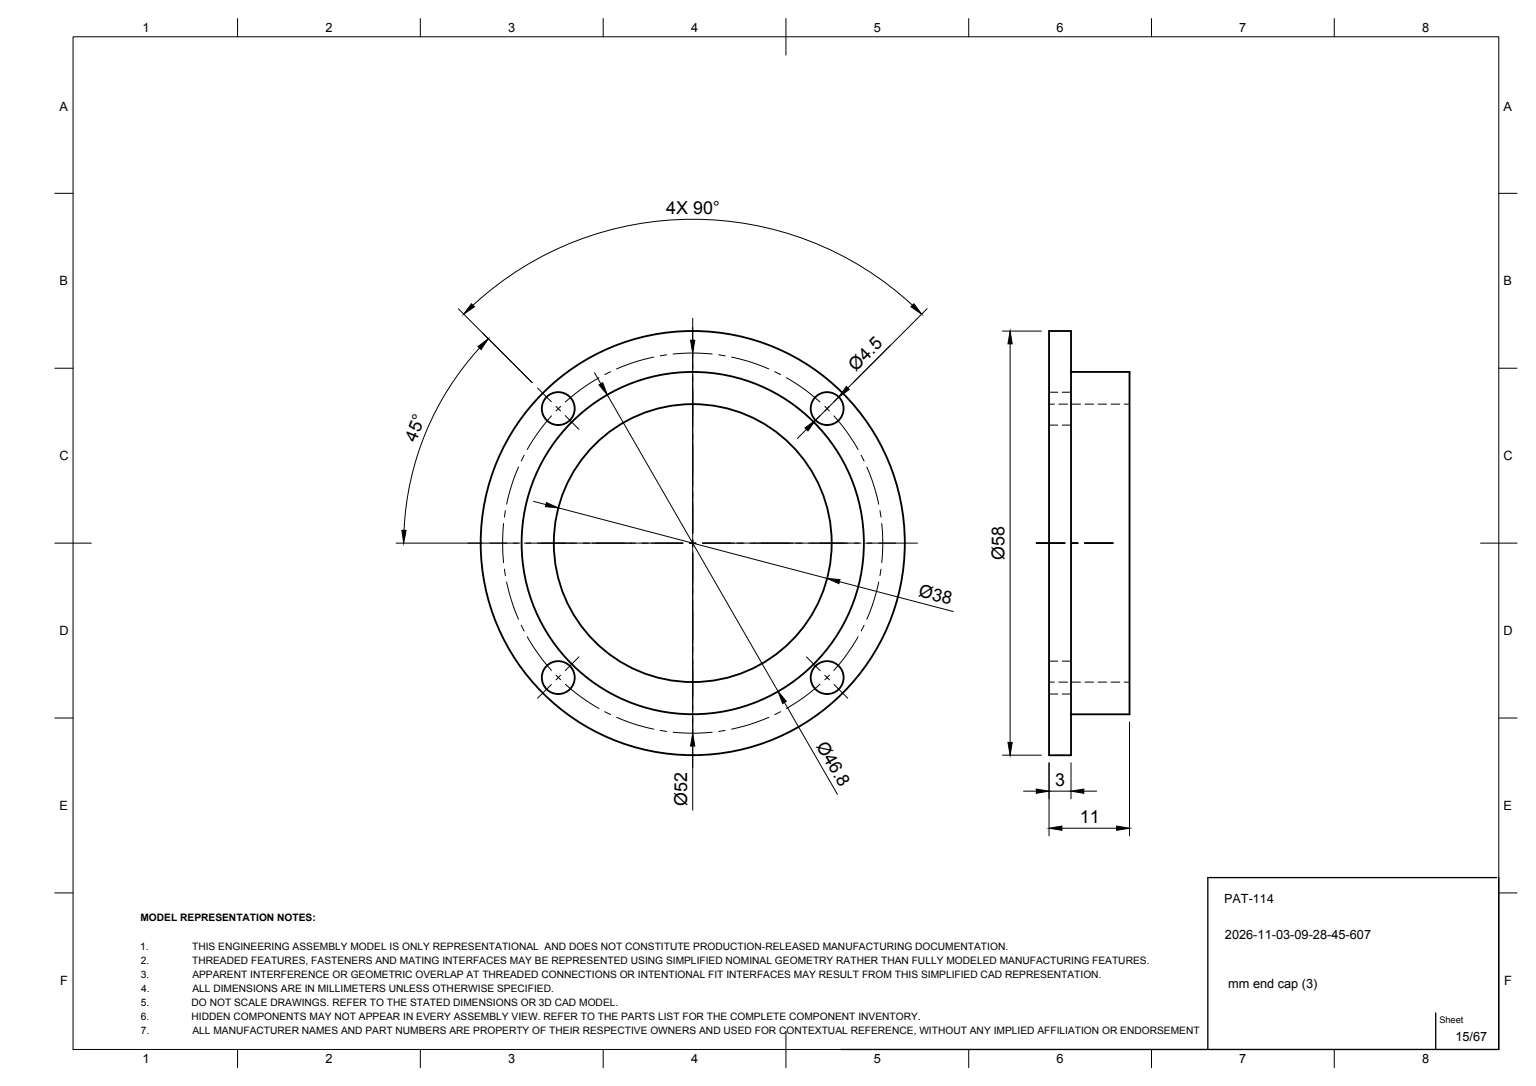
ISO-10303-21;
HEADER;
/* Generated by software containing ST-Developer
 * from STEP Tools, Inc. (www.steptools.com) 
 */

FILE_DESCRIPTION(
/* description */ ('Two-stage gear reducer in split housing'),
/* implementation_level */ '2;1');

FILE_NAME(
/* name */ 'mm end cap (3).step',
/* time_stamp */ '2026-10-28T03:22:31-07:00',
/* author */ (''),
/* organization */ (''),
/* preprocessor_version */ 'ST-DEVELOPER v20.2',
/* originating_system */ 'Autodesk Translation Framework v15.17.0.0',
/* authorisation */ '');

FILE_SCHEMA (('AUTOMOTIVE_DESIGN { 1 0 10303 214 3 1 1 }'));
ENDSEC;

DATA;
#10=MECHANICAL_DESIGN_GEOMETRIC_PRESENTATION_REPRESENTATION('',(#1244),#73366);
#1132=SHAPE_REPRESENTATION_RELATIONSHIP('SRR','None',#73619,#1188);
#1188=ADVANCED_BREP_SHAPE_REPRESENTATION('',(#1315),#73315);
#1244=STYLED_ITEM('',(#74002),#1315);
#1315=MANIFOLD_SOLID_BREP('Body1',#16132);
#1477=FACE_BOUND('',#3254,.T.);
#1478=FACE_BOUND('',#3258,.T.);
#1479=FACE_BOUND('',#3259,.T.);
#1480=FACE_BOUND('',#3260,.T.);
#1481=FACE_BOUND('',#3261,.T.);
#1482=FACE_BOUND('',#3262,.T.);
#1483=FACE_BOUND('',#3264,.T.);
#1484=FACE_BOUND('',#3265,.T.);
#1485=FACE_BOUND('',#3266,.T.);
#1486=FACE_BOUND('',#3267,.T.);
#1487=FACE_BOUND('',#3268,.T.);
#1717=PLANE('',#17300);
#1718=PLANE('',#17307);
#1719=PLANE('',#17308);
#2232=FACE_OUTER_BOUND('',#3248,.T.);
#2233=FACE_OUTER_BOUND('',#3249,.T.);
#2234=FACE_OUTER_BOUND('',#3250,.T.);
#2235=FACE_OUTER_BOUND('',#3251,.T.);
#2236=FACE_OUTER_BOUND('',#3252,.T.);
#2237=FACE_OUTER_BOUND('',#3253,.T.);
#2238=FACE_OUTER_BOUND('',#3255,.T.);
#2239=FACE_OUTER_BOUND('',#3256,.T.);
#2240=FACE_OUTER_BOUND('',#3257,.T.);
#2241=FACE_OUTER_BOUND('',#3263,.T.);
#3248=EDGE_LOOP('',(#11533,#11534,#11535,#11536));
#3249=EDGE_LOOP('',(#11537,#11538,#11539,#11540));
#3250=EDGE_LOOP('',(#11541,#11542,#11543,#11544));
#3251=EDGE_LOOP('',(#11545,#11546,#11547,#11548));
#3252=EDGE_LOOP('',(#11549,#11550,#11551,#11552));
#3253=EDGE_LOOP('',(#11553));
#3254=EDGE_LOOP('',(#11554));
#3255=EDGE_LOOP('',(#11555,#11556,#11557,#11558));
#3256=EDGE_LOOP('',(#11559,#11560,#11561,#11562));
#3257=EDGE_LOOP('',(#11563));
#3258=EDGE_LOOP('',(#11564));
#3259=EDGE_LOOP('',(#11565));
#3260=EDGE_LOOP('',(#11566));
#3261=EDGE_LOOP('',(#11567));
#3262=EDGE_LOOP('',(#11568));
#3263=EDGE_LOOP('',(#11569));
#3264=EDGE_LOOP('',(#11570));
#3265=EDGE_LOOP('',(#11571));
#3266=EDGE_LOOP('',(#11572));
#3267=EDGE_LOOP('',(#11573));
#3268=EDGE_LOOP('',(#11574));
#4339=LINE('',#23876,#5363);
#4340=LINE('',#23882,#5364);
#4341=LINE('',#23888,#5365);
#4342=LINE('',#23894,#5366);
#4343=LINE('',#23900,#5367);
#4344=LINE('',#23908,#5368);
#4345=LINE('',#23913,#5369);
#5363=VECTOR('',#19691,0.225);
#5364=VECTOR('',#19698,0.225);
#5365=VECTOR('',#19705,0.225000000000001);
#5366=VECTOR('',#19712,0.225000000000001);
#5367=VECTOR('',#19719,2.34);
#5368=VECTOR('',#19730,1.9);
#5369=VECTOR('',#19735,2.9);
#6334=CIRCLE('',#17286,0.225);
#6335=CIRCLE('',#17287,0.225);
#6336=CIRCLE('',#17289,0.225);
#6337=CIRCLE('',#17290,0.225);
#6338=CIRCLE('',#17292,0.225000000000001);
#6339=CIRCLE('',#17293,0.225000000000001);
#6340=CIRCLE('',#17295,0.225000000000001);
#6341=CIRCLE('',#17296,0.225000000000001);
#6342=CIRCLE('',#17298,2.34);
#6343=CIRCLE('',#17299,2.34);
#6344=CIRCLE('',#17301,1.9);
#6345=CIRCLE('',#17303,1.9);
#6346=CIRCLE('',#17305,2.9);
#6347=CIRCLE('',#17306,2.9);
#7166=VERTEX_POINT('',#23873);
#7167=VERTEX_POINT('',#23875);
#7168=VERTEX_POINT('',#23879);
#7169=VERTEX_POINT('',#23881);
#7170=VERTEX_POINT('',#23885);
#7171=VERTEX_POINT('',#23887);
#7172=VERTEX_POINT('',#23891);
#7173=VERTEX_POINT('',#23893);
#7174=VERTEX_POINT('',#23897);
#7175=VERTEX_POINT('',#23899);
#7176=VERTEX_POINT('',#23903);
#7177=VERTEX_POINT('',#23906);
#7178=VERTEX_POINT('',#23910);
#7179=VERTEX_POINT('',#23912);
#8820=EDGE_CURVE('',#7166,#7166,#6334,.T.);
#8821=EDGE_CURVE('',#7166,#7167,#4339,.T.);
#8822=EDGE_CURVE('',#7167,#7167,#6335,.T.);
#8823=EDGE_CURVE('',#7168,#7168,#6336,.T.);
#8824=EDGE_CURVE('',#7168,#7169,#4340,.T.);
#8825=EDGE_CURVE('',#7169,#7169,#6337,.T.);
#8826=EDGE_CURVE('',#7170,#7170,#6338,.T.);
#8827=EDGE_CURVE('',#7170,#7171,#4341,.T.);
#8828=EDGE_CURVE('',#7171,#7171,#6339,.T.);
#8829=EDGE_CURVE('',#7172,#7172,#6340,.T.);
#8830=EDGE_CURVE('',#7172,#7173,#4342,.T.);
#8831=EDGE_CURVE('',#7173,#7173,#6341,.T.);
#8832=EDGE_CURVE('',#7174,#7174,#6342,.T.);
#8833=EDGE_CURVE('',#7174,#7175,#4343,.T.);
#8834=EDGE_CURVE('',#7175,#7175,#6343,.T.);
#8835=EDGE_CURVE('',#7176,#7176,#6344,.T.);
#8836=EDGE_CURVE('',#7177,#7177,#6345,.T.);
#8837=EDGE_CURVE('',#7177,#7176,#4344,.T.);
#8838=EDGE_CURVE('',#7178,#7178,#6346,.T.);
#8839=EDGE_CURVE('',#7178,#7179,#4345,.T.);
#8840=EDGE_CURVE('',#7179,#7179,#6347,.T.);
#11533=ORIENTED_EDGE('',*,*,#8820,.F.);
#11534=ORIENTED_EDGE('',*,*,#8821,.T.);
#11535=ORIENTED_EDGE('',*,*,#8822,.F.);
#11536=ORIENTED_EDGE('',*,*,#8821,.F.);
#11537=ORIENTED_EDGE('',*,*,#8823,.F.);
#11538=ORIENTED_EDGE('',*,*,#8824,.T.);
#11539=ORIENTED_EDGE('',*,*,#8825,.F.);
#11540=ORIENTED_EDGE('',*,*,#8824,.F.);
#11541=ORIENTED_EDGE('',*,*,#8826,.F.);
#11542=ORIENTED_EDGE('',*,*,#8827,.T.);
#11543=ORIENTED_EDGE('',*,*,#8828,.F.);
#11544=ORIENTED_EDGE('',*,*,#8827,.F.);
#11545=ORIENTED_EDGE('',*,*,#8829,.F.);
#11546=ORIENTED_EDGE('',*,*,#8830,.T.);
#11547=ORIENTED_EDGE('',*,*,#8831,.F.);
#11548=ORIENTED_EDGE('',*,*,#8830,.F.);
#11549=ORIENTED_EDGE('',*,*,#8832,.F.);
#11550=ORIENTED_EDGE('',*,*,#8833,.T.);
#11551=ORIENTED_EDGE('',*,*,#8834,.T.);
#11552=ORIENTED_EDGE('',*,*,#8833,.F.);
#11553=ORIENTED_EDGE('',*,*,#8834,.F.);
#11554=ORIENTED_EDGE('',*,*,#8835,.F.);
#11555=ORIENTED_EDGE('',*,*,#8836,.F.);
#11556=ORIENTED_EDGE('',*,*,#8837,.T.);
#11557=ORIENTED_EDGE('',*,*,#8835,.T.);
#11558=ORIENTED_EDGE('',*,*,#8837,.F.);
#11559=ORIENTED_EDGE('',*,*,#8838,.F.);
#11560=ORIENTED_EDGE('',*,*,#8839,.T.);
#11561=ORIENTED_EDGE('',*,*,#8840,.T.);
#11562=ORIENTED_EDGE('',*,*,#8839,.F.);
#11563=ORIENTED_EDGE('',*,*,#8838,.T.);
#11564=ORIENTED_EDGE('',*,*,#8836,.T.);
#11565=ORIENTED_EDGE('',*,*,#8831,.T.);
#11566=ORIENTED_EDGE('',*,*,#8828,.T.);
#11567=ORIENTED_EDGE('',*,*,#8825,.T.);
#11568=ORIENTED_EDGE('',*,*,#8822,.T.);
#11569=ORIENTED_EDGE('',*,*,#8840,.F.);
#11570=ORIENTED_EDGE('',*,*,#8832,.T.);
#11571=ORIENTED_EDGE('',*,*,#8829,.T.);
#11572=ORIENTED_EDGE('',*,*,#8826,.T.);
#11573=ORIENTED_EDGE('',*,*,#8823,.T.);
#11574=ORIENTED_EDGE('',*,*,#8820,.T.);
#15022=CYLINDRICAL_SURFACE('',#17285,0.225);
#15023=CYLINDRICAL_SURFACE('',#17288,0.225);
#15024=CYLINDRICAL_SURFACE('',#17291,0.225000000000001);
#15025=CYLINDRICAL_SURFACE('',#17294,0.225000000000001);
#15026=CYLINDRICAL_SURFACE('',#17297,2.34);
#15027=CYLINDRICAL_SURFACE('',#17302,1.9);
#15028=CYLINDRICAL_SURFACE('',#17304,2.9);
#15439=ADVANCED_FACE('',(#2232),#15022,.F.);
#15440=ADVANCED_FACE('',(#2233),#15023,.F.);
#15441=ADVANCED_FACE('',(#2234),#15024,.F.);
#15442=ADVANCED_FACE('',(#2235),#15025,.F.);
#15443=ADVANCED_FACE('',(#2236),#15026,.T.);
#15444=ADVANCED_FACE('',(#2237,#1477),#1717,.F.);
#15445=ADVANCED_FACE('',(#2238),#15027,.F.);
#15446=ADVANCED_FACE('',(#2239),#15028,.T.);
#15447=ADVANCED_FACE('',(#2240,#1478,#1479,#1480,#1481,#1482),#1718,.T.);
#15448=ADVANCED_FACE('',(#2241,#1483,#1484,#1485,#1486,#1487),#1719,.F.);
#16132=CLOSED_SHELL('',(#15439,#15440,#15441,#15442,#15443,#15444,#15445,
#15446,#15447,#15448));
#17284=AXIS2_PLACEMENT_3D('',#23871,#19685,#19686);
#17285=AXIS2_PLACEMENT_3D('',#23872,#19687,#19688);
#17286=AXIS2_PLACEMENT_3D('',#23874,#19689,#19690);
#17287=AXIS2_PLACEMENT_3D('',#23877,#19692,#19693);
#17288=AXIS2_PLACEMENT_3D('',#23878,#19694,#19695);
#17289=AXIS2_PLACEMENT_3D('',#23880,#19696,#19697);
#17290=AXIS2_PLACEMENT_3D('',#23883,#19699,#19700);
#17291=AXIS2_PLACEMENT_3D('',#23884,#19701,#19702);
#17292=AXIS2_PLACEMENT_3D('',#23886,#19703,#19704);
#17293=AXIS2_PLACEMENT_3D('',#23889,#19706,#19707);
#17294=AXIS2_PLACEMENT_3D('',#23890,#19708,#19709);
#17295=AXIS2_PLACEMENT_3D('',#23892,#19710,#19711);
#17296=AXIS2_PLACEMENT_3D('',#23895,#19713,#19714);
#17297=AXIS2_PLACEMENT_3D('',#23896,#19715,#19716);
#17298=AXIS2_PLACEMENT_3D('',#23898,#19717,#19718);
#17299=AXIS2_PLACEMENT_3D('',#23901,#19720,#19721);
#17300=AXIS2_PLACEMENT_3D('',#23902,#19722,#19723);
#17301=AXIS2_PLACEMENT_3D('',#23904,#19724,#19725);
#17302=AXIS2_PLACEMENT_3D('',#23905,#19726,#19727);
#17303=AXIS2_PLACEMENT_3D('',#23907,#19728,#19729);
#17304=AXIS2_PLACEMENT_3D('',#23909,#19731,#19732);
#17305=AXIS2_PLACEMENT_3D('',#23911,#19733,#19734);
#17306=AXIS2_PLACEMENT_3D('',#23914,#19736,#19737);
#17307=AXIS2_PLACEMENT_3D('',#23915,#19738,#19739);
#17308=AXIS2_PLACEMENT_3D('',#23916,#19740,#19741);
#19685=DIRECTION('axis',(0.,0.,1.));
#19686=DIRECTION('refdir',(1.,0.,0.));
#19687=DIRECTION('center_axis',(0.,1.,0.));
#19688=DIRECTION('ref_axis',(1.,0.,0.));
#19689=DIRECTION('center_axis',(0.,1.,0.));
#19690=DIRECTION('ref_axis',(1.,0.,0.));
#19691=DIRECTION('',(0.,1.,0.));
#19692=DIRECTION('center_axis',(0.,-1.,0.));
#19693=DIRECTION('ref_axis',(1.,0.,0.));
#19694=DIRECTION('center_axis',(0.,1.,0.));
#19695=DIRECTION('ref_axis',(1.,0.,0.));
#19696=DIRECTION('center_axis',(0.,1.,0.));
#19697=DIRECTION('ref_axis',(1.,0.,0.));
#19698=DIRECTION('',(0.,1.,0.));
#19699=DIRECTION('center_axis',(0.,-1.,0.));
#19700=DIRECTION('ref_axis',(1.,0.,0.));
#19701=DIRECTION('center_axis',(0.,1.,0.));
#19702=DIRECTION('ref_axis',(1.,0.,0.));
#19703=DIRECTION('center_axis',(0.,1.,0.));
#19704=DIRECTION('ref_axis',(1.,0.,0.));
#19705=DIRECTION('',(0.,1.,0.));
#19706=DIRECTION('center_axis',(0.,-1.,0.));
#19707=DIRECTION('ref_axis',(1.,0.,0.));
#19708=DIRECTION('center_axis',(0.,1.,0.));
#19709=DIRECTION('ref_axis',(1.,0.,0.));
#19710=DIRECTION('center_axis',(0.,1.,0.));
#19711=DIRECTION('ref_axis',(1.,0.,0.));
#19712=DIRECTION('',(0.,1.,0.));
#19713=DIRECTION('center_axis',(0.,-1.,0.));
#19714=DIRECTION('ref_axis',(1.,0.,0.));
#19715=DIRECTION('center_axis',(0.,1.,0.));
#19716=DIRECTION('ref_axis',(1.,0.,0.));
#19717=DIRECTION('center_axis',(0.,1.,0.));
#19718=DIRECTION('ref_axis',(1.,0.,0.));
#19719=DIRECTION('',(0.,-1.,0.));
#19720=DIRECTION('center_axis',(0.,1.,0.));
#19721=DIRECTION('ref_axis',(1.,0.,0.));
#19722=DIRECTION('center_axis',(0.,1.,0.));
#19723=DIRECTION('ref_axis',(1.,0.,0.));
#19724=DIRECTION('center_axis',(0.,-1.,0.));
#19725=DIRECTION('ref_axis',(1.,0.,0.));
#19726=DIRECTION('center_axis',(0.,1.,0.));
#19727=DIRECTION('ref_axis',(1.,0.,0.));
#19728=DIRECTION('center_axis',(0.,-1.,0.));
#19729=DIRECTION('ref_axis',(1.,0.,0.));
#19730=DIRECTION('',(0.,-1.,0.));
#19731=DIRECTION('center_axis',(0.,1.,0.));
#19732=DIRECTION('ref_axis',(1.,0.,0.));
#19733=DIRECTION('center_axis',(0.,1.,0.));
#19734=DIRECTION('ref_axis',(1.,0.,0.));
#19735=DIRECTION('',(0.,-1.,0.));
#19736=DIRECTION('center_axis',(0.,1.,0.));
#19737=DIRECTION('ref_axis',(1.,0.,0.));
#19738=DIRECTION('center_axis',(0.,1.,0.));
#19739=DIRECTION('ref_axis',(1.,0.,0.));
#19740=DIRECTION('center_axis',(0.,1.,0.));
#19741=DIRECTION('ref_axis',(1.,0.,0.));
#23871=CARTESIAN_POINT('',(0.,0.,0.));
#23872=CARTESIAN_POINT('Origin',(4.16152236891498,7.4,8.16152236891498));
#23873=CARTESIAN_POINT('',(3.93652236891498,7.5,8.16152236891498));
#23874=CARTESIAN_POINT('Origin',(4.16152236891498,7.5,8.16152236891498));
#23875=CARTESIAN_POINT('',(3.93652236891498,7.8,8.16152236891498));
#23876=CARTESIAN_POINT('',(3.93652236891498,7.4,8.16152236891498));
#23877=CARTESIAN_POINT('Origin',(4.16152236891498,7.8,8.16152236891498));
#23878=CARTESIAN_POINT('Origin',(4.16152236891498,7.4,11.838477631085));
#23879=CARTESIAN_POINT('',(3.93652236891498,7.5,11.838477631085));
#23880=CARTESIAN_POINT('Origin',(4.16152236891498,7.5,11.838477631085));
#23881=CARTESIAN_POINT('',(3.93652236891498,7.8,11.838477631085));
#23882=CARTESIAN_POINT('',(3.93652236891498,7.4,11.838477631085));
#23883=CARTESIAN_POINT('Origin',(4.16152236891498,7.8,11.838477631085));
#23884=CARTESIAN_POINT('Origin',(7.83847763108502,7.4,11.838477631085));
#23885=CARTESIAN_POINT('',(7.61347763108502,7.5,11.838477631085));
#23886=CARTESIAN_POINT('Origin',(7.83847763108502,7.5,11.838477631085));
#23887=CARTESIAN_POINT('',(7.61347763108502,7.8,11.838477631085));
#23888=CARTESIAN_POINT('',(7.61347763108502,7.4,11.838477631085));
#23889=CARTESIAN_POINT('Origin',(7.83847763108502,7.8,11.838477631085));
#23890=CARTESIAN_POINT('Origin',(7.83847763108502,7.4,8.16152236891498));
#23891=CARTESIAN_POINT('',(7.61347763108502,7.5,8.16152236891498));
#23892=CARTESIAN_POINT('Origin',(7.83847763108502,7.5,8.16152236891498));
#23893=CARTESIAN_POINT('',(7.61347763108502,7.8,8.16152236891498));
#23894=CARTESIAN_POINT('',(7.61347763108502,7.4,8.16152236891498));
#23895=CARTESIAN_POINT('Origin',(7.83847763108502,7.8,8.16152236891498));
#23896=CARTESIAN_POINT('Origin',(6.,6.7,10.));
#23897=CARTESIAN_POINT('',(3.66,7.5,10.));
#23898=CARTESIAN_POINT('Origin',(6.,7.5,10.));
#23899=CARTESIAN_POINT('',(3.66,6.7,10.));
#23900=CARTESIAN_POINT('',(3.66,6.7,10.));
#23901=CARTESIAN_POINT('Origin',(6.,6.7,10.));
#23902=CARTESIAN_POINT('Origin',(6.,6.7,10.));
#23903=CARTESIAN_POINT('',(4.1,6.7,10.));
#23904=CARTESIAN_POINT('Origin',(6.,6.7,10.));
#23905=CARTESIAN_POINT('Origin',(6.,7.5,10.));
#23906=CARTESIAN_POINT('',(4.1,7.8,10.));
#23907=CARTESIAN_POINT('Origin',(6.,7.8,10.));
#23908=CARTESIAN_POINT('',(4.1,7.5,10.));
#23909=CARTESIAN_POINT('Origin',(6.,7.5,10.));
#23910=CARTESIAN_POINT('',(3.1,7.8,10.));
#23911=CARTESIAN_POINT('Origin',(6.,7.8,10.));
#23912=CARTESIAN_POINT('',(3.1,7.5,10.));
#23913=CARTESIAN_POINT('',(3.1,7.5,10.));
#23914=CARTESIAN_POINT('Origin',(6.,7.5,10.));
#23915=CARTESIAN_POINT('Origin',(6.,7.8,10.));
#23916=CARTESIAN_POINT('Origin',(6.,7.5,10.));
#73251=UNCERTAINTY_MEASURE_WITH_UNIT(LENGTH_MEASURE(0.001),#73367,
'DISTANCE_ACCURACY_VALUE',
'Maximum model space distance between geometric entities at asserted c
onnectivities');
#73302=UNCERTAINTY_MEASURE_WITH_UNIT(LENGTH_MEASURE(0.001),#73367,
'DISTANCE_ACCURACY_VALUE',
'Maximum model space distance between geometric entities at asserted c
onnectivities');
#73315=(
GEOMETRIC_REPRESENTATION_CONTEXT(3)
GLOBAL_UNCERTAINTY_ASSIGNED_CONTEXT((#73251))
GLOBAL_UNIT_ASSIGNED_CONTEXT((#73367,#73369,#73370))
REPRESENTATION_CONTEXT('','3D')
);
#73366=(
GEOMETRIC_REPRESENTATION_CONTEXT(3)
GLOBAL_UNCERTAINTY_ASSIGNED_CONTEXT((#73302))
GLOBAL_UNIT_ASSIGNED_CONTEXT((#73367,#73369,#73370))
REPRESENTATION_CONTEXT('','3D')
);
#73367=(
LENGTH_UNIT()
NAMED_UNIT(*)
SI_UNIT(.CENTI.,.METRE.)
);
#73369=(
NAMED_UNIT(*)
PLANE_ANGLE_UNIT()
SI_UNIT($,.RADIAN.)
);
#73370=(
NAMED_UNIT(*)
SI_UNIT($,.STERADIAN.)
SOLID_ANGLE_UNIT()
);
#73383=SHAPE_DEFINITION_REPRESENTATION(#73446,#73619);
#73446=PRODUCT_DEFINITION_SHAPE('',$,#73683);
#73619=SHAPE_REPRESENTATION('',(#17284),#73315);
#73670=PRODUCT_DEFINITION_CONTEXT('part definition',#73861,'design');
#73683=PRODUCT_DEFINITION('mm end cap (3)','mm end cap (3)',#73746,#73670);
#73746=PRODUCT_DEFINITION_FORMATION('',$,#73875);
#73861=APPLICATION_CONTEXT(
'Core Data for Automotive Mechanical Design Process');
#73862=PRODUCT_CONTEXT('part definition',#73861,'mechanical');
#73875=PRODUCT('mm end cap (3)','mm end cap (3)','mm end cap (3)',(#73862));
#73996=COLOUR_RGB('Off White',0.89,0.88,0.83);
#73997=FILL_AREA_STYLE_COLOUR('',#73996);
#73998=FILL_AREA_STYLE('',(#73997));
#73999=SURFACE_STYLE_FILL_AREA(#73998);
#74000=SURFACE_SIDE_STYLE('',(#73999));
#74001=SURFACE_STYLE_USAGE(.BOTH.,#74000);
#74002=PRESENTATION_STYLE_ASSIGNMENT((#74001));
ENDSEC;
END-ISO-10303-21;
